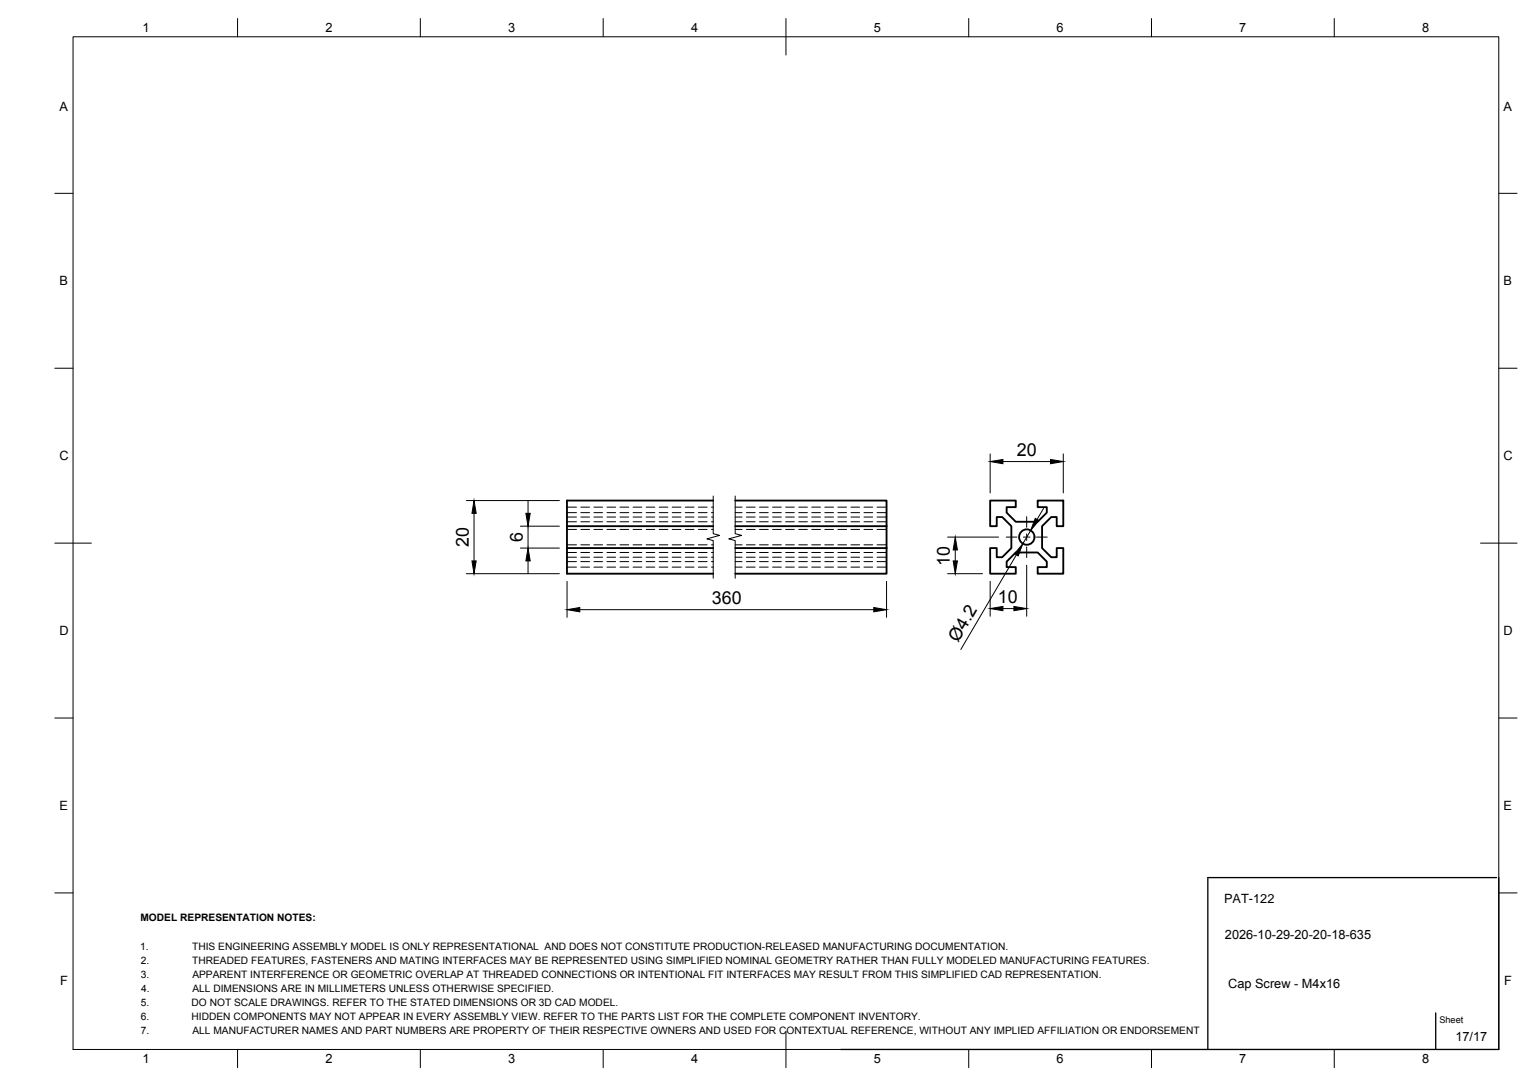
ISO-10303-21;
HEADER;
/* Generated by software containing ST-Developer
 * from STEP Tools, Inc. (www.steptools.com) 
 */

FILE_DESCRIPTION(
/* description */ ('PAT-122'),
/* implementation_level */ '2;1');

FILE_NAME(
/* name */ 'Cap Screw - M4x16.step',
/* time_stamp */ '2026-10-29T20:20:12-07:00',
/* author */ (''),
/* organization */ (''),
/* preprocessor_version */ 'ST-DEVELOPER v20.2',
/* originating_system */ 'Autodesk Translation Framework v15.17.0.0',
/* authorisation */ '');

FILE_SCHEMA (('AUTOMOTIVE_DESIGN { 1 0 10303 214 3 1 1 }'));
ENDSEC;

DATA;
#10=MECHANICAL_DESIGN_GEOMETRIC_PRESENTATION_REPRESENTATION('',(#512),#10019);
#413=CONICAL_SURFACE('',#6306,0.325,0.785398163397448);
#414=CONICAL_SURFACE('',#6310,0.335,0.785398163397448);
#415=CONICAL_SURFACE('',#6314,0.21,0.463647609000806);
#416=CONICAL_SURFACE('',#6318,0.18,0.785398163397448);
#420=ORIENTED_CLOSED_SHELL('',*,#5638,.F.);
#424=BREP_WITH_VOIDS('Body1',#5637,(#420));
#468=SHAPE_REPRESENTATION_RELATIONSHIP('SRR','None',#10189,#490);
#490=ADVANCED_BREP_SHAPE_REPRESENTATION('',(#424),#10018);
#512=STYLED_ITEM('',(#10355),#424);
#608=FACE_BOUND('',#1474,.T.);
#814=PLANE('',#6304);
#815=PLANE('',#6312);
#816=PLANE('',#6320);
#817=PLANE('',#6321);
#818=PLANE('',#6322);
#819=PLANE('',#6323);
#820=PLANE('',#6324);
#821=PLANE('',#6325);
#822=PLANE('',#6326);
#823=PLANE('',#6327);
#824=PLANE('',#6328);
#1100=FACE_OUTER_BOUND('',#1469,.T.);
#1101=FACE_OUTER_BOUND('',#1470,.T.);
#1102=FACE_OUTER_BOUND('',#1471,.T.);
#1103=FACE_OUTER_BOUND('',#1472,.T.);
#1104=FACE_OUTER_BOUND('',#1473,.T.);
#1105=FACE_OUTER_BOUND('',#1475,.T.);
#1106=FACE_OUTER_BOUND('',#1476,.T.);
#1107=FACE_OUTER_BOUND('',#1477,.T.);
#1108=FACE_OUTER_BOUND('',#1478,.T.);
#1109=FACE_OUTER_BOUND('',#1479,.T.);
#1110=FACE_OUTER_BOUND('',#1480,.T.);
#1111=FACE_OUTER_BOUND('',#1481,.T.);
#1112=FACE_OUTER_BOUND('',#1482,.T.);
#1113=FACE_OUTER_BOUND('',#1483,.T.);
#1114=FACE_OUTER_BOUND('',#1484,.T.);
#1115=FACE_OUTER_BOUND('',#1485,.T.);
#1116=FACE_OUTER_BOUND('',#1486,.T.);
#1469=EDGE_LOOP('',(#5197));
#1470=EDGE_LOOP('',(#5198,#5199,#5200,#5201));
#1471=EDGE_LOOP('',(#5202,#5203,#5204,#5205));
#1472=EDGE_LOOP('',(#5206,#5207,#5208,#5209));
#1473=EDGE_LOOP('',(#5210));
#1474=EDGE_LOOP('',(#5211));
#1475=EDGE_LOOP('',(#5212,#5213,#5214,#5215));
#1476=EDGE_LOOP('',(#5216,#5217,#5218,#5219));
#1477=EDGE_LOOP('',(#5220,#5221,#5222,#5223));
#1478=EDGE_LOOP('',(#5224));
#1479=EDGE_LOOP('',(#5225,#5226,#5227,#5228));
#1480=EDGE_LOOP('',(#5229,#5230,#5231,#5232));
#1481=EDGE_LOOP('',(#5233,#5234,#5235,#5236));
#1482=EDGE_LOOP('',(#5237,#5238,#5239,#5240));
#1483=EDGE_LOOP('',(#5241,#5242,#5243,#5244));
#1484=EDGE_LOOP('',(#5245,#5246,#5247,#5248));
#1485=EDGE_LOOP('',(#5249,#5250,#5251,#5252,#5253,#5254));
#1486=EDGE_LOOP('',(#5255,#5256,#5257,#5258,#5259,#5260));
#2007=LINE('',#9812,#2551);
#2008=LINE('',#9816,#2552);
#2009=LINE('',#9820,#2553);
#2010=LINE('',#9827,#2554);
#2011=LINE('',#9831,#2555);
#2012=LINE('',#9835,#2556);
#2013=LINE('',#9840,#2557);
#2014=LINE('',#9842,#2558);
#2015=LINE('',#9844,#2559);
#2016=LINE('',#9845,#2560);
#2017=LINE('',#9848,#2561);
#2018=LINE('',#9850,#2562);
#2019=LINE('',#9851,#2563);
#2020=LINE('',#9854,#2564);
#2021=LINE('',#9856,#2565);
#2022=LINE('',#9857,#2566);
#2023=LINE('',#9860,#2567);
#2024=LINE('',#9862,#2568);
#2025=LINE('',#9863,#2569);
#2026=LINE('',#9866,#2570);
#2027=LINE('',#9868,#2571);
#2028=LINE('',#9869,#2572);
#2029=LINE('',#9871,#2573);
#2030=LINE('',#9872,#2574);
#2551=VECTOR('',#7798,0.325);
#2552=VECTOR('',#7803,0.35);
#2553=VECTOR('',#7808,0.335);
#2554=VECTOR('',#7817,0.21);
#2555=VECTOR('',#7822,0.2);
#2556=VECTOR('',#7827,0.18);
#2557=VECTOR('',#7832,1.);
#2558=VECTOR('',#7833,1.);
#2559=VECTOR('',#7834,1.);
#2560=VECTOR('',#7835,1.);
#2561=VECTOR('',#7838,1.);
#2562=VECTOR('',#7839,1.);
#2563=VECTOR('',#7840,1.);
#2564=VECTOR('',#7843,1.);
#2565=VECTOR('',#7844,1.);
#2566=VECTOR('',#7845,1.);
#2567=VECTOR('',#7848,1.);
#2568=VECTOR('',#7849,1.);
#2569=VECTOR('',#7850,1.);
#2570=VECTOR('',#7853,1.);
#2571=VECTOR('',#7854,1.);
#2572=VECTOR('',#7855,1.);
#2573=VECTOR('',#7858,1.);
#2574=VECTOR('',#7859,1.);
#2697=CIRCLE('',#6305,0.3);
#2698=CIRCLE('',#6307,0.35);
#2699=CIRCLE('',#6309,0.35);
#2700=CIRCLE('',#6311,0.32);
#2701=CIRCLE('',#6313,0.22);
#2702=CIRCLE('',#6315,0.1954);
#2703=CIRCLE('',#6317,0.1954);
#2704=CIRCLE('',#6319,0.16);
#3147=VERTEX_POINT('',#9807);
#3148=VERTEX_POINT('',#9810);
#3149=VERTEX_POINT('',#9814);
#3150=VERTEX_POINT('',#9818);
#3151=VERTEX_POINT('',#9822);
#3152=VERTEX_POINT('',#9825);
#3153=VERTEX_POINT('',#9829);
#3154=VERTEX_POINT('',#9833);
#3155=VERTEX_POINT('',#9838);
#3156=VERTEX_POINT('',#9839);
#3157=VERTEX_POINT('',#9841);
#3158=VERTEX_POINT('',#9843);
#3159=VERTEX_POINT('',#9847);
#3160=VERTEX_POINT('',#9849);
#3161=VERTEX_POINT('',#9853);
#3162=VERTEX_POINT('',#9855);
#3163=VERTEX_POINT('',#9859);
#3164=VERTEX_POINT('',#9861);
#3165=VERTEX_POINT('',#9865);
#3166=VERTEX_POINT('',#9867);
#3833=EDGE_CURVE('',#3147,#3147,#2697,.T.);
#3834=EDGE_CURVE('',#3148,#3148,#2698,.T.);
#3835=EDGE_CURVE('',#3148,#3147,#2007,.T.);
#3836=EDGE_CURVE('',#3149,#3149,#2699,.T.);
#3837=EDGE_CURVE('',#3149,#3148,#2008,.T.);
#3838=EDGE_CURVE('',#3150,#3150,#2700,.T.);
#3839=EDGE_CURVE('',#3150,#3149,#2009,.T.);
#3840=EDGE_CURVE('',#3151,#3151,#2701,.T.);
#3841=EDGE_CURVE('',#3152,#3152,#2702,.F.);
#3842=EDGE_CURVE('',#3152,#3151,#2010,.T.);
#3843=EDGE_CURVE('',#3153,#3153,#2703,.F.);
#3844=EDGE_CURVE('',#3153,#3152,#2011,.T.);
#3845=EDGE_CURVE('',#3154,#3154,#2704,.T.);
#3846=EDGE_CURVE('',#3154,#3153,#2012,.T.);
#3847=EDGE_CURVE('',#3155,#3156,#2013,.T.);
#3848=EDGE_CURVE('',#3156,#3157,#2014,.T.);
#3849=EDGE_CURVE('',#3157,#3158,#2015,.T.);
#3850=EDGE_CURVE('',#3155,#3158,#2016,.T.);
#3851=EDGE_CURVE('',#3156,#3159,#2017,.T.);
#3852=EDGE_CURVE('',#3159,#3160,#2018,.T.);
#3853=EDGE_CURVE('',#3160,#3157,#2019,.T.);
#3854=EDGE_CURVE('',#3159,#3161,#2020,.T.);
#3855=EDGE_CURVE('',#3161,#3162,#2021,.T.);
#3856=EDGE_CURVE('',#3162,#3160,#2022,.T.);
#3857=EDGE_CURVE('',#3161,#3163,#2023,.T.);
#3858=EDGE_CURVE('',#3163,#3164,#2024,.T.);
#3859=EDGE_CURVE('',#3164,#3162,#2025,.T.);
#3860=EDGE_CURVE('',#3163,#3165,#2026,.T.);
#3861=EDGE_CURVE('',#3165,#3166,#2027,.T.);
#3862=EDGE_CURVE('',#3166,#3164,#2028,.T.);
#3863=EDGE_CURVE('',#3165,#3155,#2029,.T.);
#3864=EDGE_CURVE('',#3158,#3166,#2030,.T.);
#5197=ORIENTED_EDGE('',*,*,#3833,.F.);
#5198=ORIENTED_EDGE('',*,*,#3834,.F.);
#5199=ORIENTED_EDGE('',*,*,#3835,.T.);
#5200=ORIENTED_EDGE('',*,*,#3833,.T.);
#5201=ORIENTED_EDGE('',*,*,#3835,.F.);
#5202=ORIENTED_EDGE('',*,*,#3836,.F.);
#5203=ORIENTED_EDGE('',*,*,#3837,.T.);
#5204=ORIENTED_EDGE('',*,*,#3834,.T.);
#5205=ORIENTED_EDGE('',*,*,#3837,.F.);
#5206=ORIENTED_EDGE('',*,*,#3838,.F.);
#5207=ORIENTED_EDGE('',*,*,#3839,.T.);
#5208=ORIENTED_EDGE('',*,*,#3836,.T.);
#5209=ORIENTED_EDGE('',*,*,#3839,.F.);
#5210=ORIENTED_EDGE('',*,*,#3838,.T.);
#5211=ORIENTED_EDGE('',*,*,#3840,.F.);
#5212=ORIENTED_EDGE('',*,*,#3841,.F.);
#5213=ORIENTED_EDGE('',*,*,#3842,.T.);
#5214=ORIENTED_EDGE('',*,*,#3840,.T.);
#5215=ORIENTED_EDGE('',*,*,#3842,.F.);
#5216=ORIENTED_EDGE('',*,*,#3843,.F.);
#5217=ORIENTED_EDGE('',*,*,#3844,.T.);
#5218=ORIENTED_EDGE('',*,*,#3841,.T.);
#5219=ORIENTED_EDGE('',*,*,#3844,.F.);
#5220=ORIENTED_EDGE('',*,*,#3845,.F.);
#5221=ORIENTED_EDGE('',*,*,#3846,.T.);
#5222=ORIENTED_EDGE('',*,*,#3843,.T.);
#5223=ORIENTED_EDGE('',*,*,#3846,.F.);
#5224=ORIENTED_EDGE('',*,*,#3845,.T.);
#5225=ORIENTED_EDGE('',*,*,#3847,.T.);
#5226=ORIENTED_EDGE('',*,*,#3848,.T.);
#5227=ORIENTED_EDGE('',*,*,#3849,.T.);
#5228=ORIENTED_EDGE('',*,*,#3850,.F.);
#5229=ORIENTED_EDGE('',*,*,#3851,.T.);
#5230=ORIENTED_EDGE('',*,*,#3852,.T.);
#5231=ORIENTED_EDGE('',*,*,#3853,.T.);
#5232=ORIENTED_EDGE('',*,*,#3848,.F.);
#5233=ORIENTED_EDGE('',*,*,#3854,.T.);
#5234=ORIENTED_EDGE('',*,*,#3855,.T.);
#5235=ORIENTED_EDGE('',*,*,#3856,.T.);
#5236=ORIENTED_EDGE('',*,*,#3852,.F.);
#5237=ORIENTED_EDGE('',*,*,#3857,.T.);
#5238=ORIENTED_EDGE('',*,*,#3858,.T.);
#5239=ORIENTED_EDGE('',*,*,#3859,.T.);
#5240=ORIENTED_EDGE('',*,*,#3855,.F.);
#5241=ORIENTED_EDGE('',*,*,#3860,.T.);
#5242=ORIENTED_EDGE('',*,*,#3861,.T.);
#5243=ORIENTED_EDGE('',*,*,#3862,.T.);
#5244=ORIENTED_EDGE('',*,*,#3858,.F.);
#5245=ORIENTED_EDGE('',*,*,#3863,.T.);
#5246=ORIENTED_EDGE('',*,*,#3850,.T.);
#5247=ORIENTED_EDGE('',*,*,#3864,.T.);
#5248=ORIENTED_EDGE('',*,*,#3861,.F.);
#5249=ORIENTED_EDGE('',*,*,#3863,.F.);
#5250=ORIENTED_EDGE('',*,*,#3860,.F.);
#5251=ORIENTED_EDGE('',*,*,#3857,.F.);
#5252=ORIENTED_EDGE('',*,*,#3854,.F.);
#5253=ORIENTED_EDGE('',*,*,#3851,.F.);
#5254=ORIENTED_EDGE('',*,*,#3847,.F.);
#5255=ORIENTED_EDGE('',*,*,#3864,.F.);
#5256=ORIENTED_EDGE('',*,*,#3849,.F.);
#5257=ORIENTED_EDGE('',*,*,#3853,.F.);
#5258=ORIENTED_EDGE('',*,*,#3856,.F.);
#5259=ORIENTED_EDGE('',*,*,#3859,.F.);
#5260=ORIENTED_EDGE('',*,*,#3862,.F.);
#5319=CYLINDRICAL_SURFACE('',#6308,0.35);
#5320=CYLINDRICAL_SURFACE('',#6316,0.1954);
#5596=ADVANCED_FACE('',(#1100),#814,.T.);
#5597=ADVANCED_FACE('',(#1101),#413,.T.);
#5598=ADVANCED_FACE('',(#1102),#5319,.T.);
#5599=ADVANCED_FACE('',(#1103),#414,.T.);
#5600=ADVANCED_FACE('',(#1104,#608),#815,.T.);
#5601=ADVANCED_FACE('',(#1105),#415,.T.);
#5602=ADVANCED_FACE('',(#1106),#5320,.T.);
#5603=ADVANCED_FACE('',(#1107),#416,.T.);
#5604=ADVANCED_FACE('',(#1108),#816,.T.);
#5605=ADVANCED_FACE('',(#1109),#817,.F.);
#5606=ADVANCED_FACE('',(#1110),#818,.F.);
#5607=ADVANCED_FACE('',(#1111),#819,.F.);
#5608=ADVANCED_FACE('',(#1112),#820,.F.);
#5609=ADVANCED_FACE('',(#1113),#821,.F.);
#5610=ADVANCED_FACE('',(#1114),#822,.F.);
#5611=ADVANCED_FACE('',(#1115),#823,.F.);
#5612=ADVANCED_FACE('',(#1116),#824,.F.);
#5637=CLOSED_SHELL('',(#5596,#5597,#5598,#5599,#5600,#5601,#5602,#5603,
#5604));
#5638=CLOSED_SHELL('',(#5605,#5606,#5607,#5608,#5609,#5610,#5611,#5612));
#6303=AXIS2_PLACEMENT_3D('',#9805,#7788,#7789);
#6304=AXIS2_PLACEMENT_3D('',#9806,#7790,#7791);
#6305=AXIS2_PLACEMENT_3D('',#9808,#7792,#7793);
#6306=AXIS2_PLACEMENT_3D('',#9809,#7794,#7795);
#6307=AXIS2_PLACEMENT_3D('',#9811,#7796,#7797);
#6308=AXIS2_PLACEMENT_3D('',#9813,#7799,#7800);
#6309=AXIS2_PLACEMENT_3D('',#9815,#7801,#7802);
#6310=AXIS2_PLACEMENT_3D('',#9817,#7804,#7805);
#6311=AXIS2_PLACEMENT_3D('',#9819,#7806,#7807);
#6312=AXIS2_PLACEMENT_3D('',#9821,#7809,#7810);
#6313=AXIS2_PLACEMENT_3D('',#9823,#7811,#7812);
#6314=AXIS2_PLACEMENT_3D('',#9824,#7813,#7814);
#6315=AXIS2_PLACEMENT_3D('',#9826,#7815,#7816);
#6316=AXIS2_PLACEMENT_3D('',#9828,#7818,#7819);
#6317=AXIS2_PLACEMENT_3D('',#9830,#7820,#7821);
#6318=AXIS2_PLACEMENT_3D('',#9832,#7823,#7824);
#6319=AXIS2_PLACEMENT_3D('',#9834,#7825,#7826);
#6320=AXIS2_PLACEMENT_3D('',#9836,#7828,#7829);
#6321=AXIS2_PLACEMENT_3D('',#9837,#7830,#7831);
#6322=AXIS2_PLACEMENT_3D('',#9846,#7836,#7837);
#6323=AXIS2_PLACEMENT_3D('',#9852,#7841,#7842);
#6324=AXIS2_PLACEMENT_3D('',#9858,#7846,#7847);
#6325=AXIS2_PLACEMENT_3D('',#9864,#7851,#7852);
#6326=AXIS2_PLACEMENT_3D('',#9870,#7856,#7857);
#6327=AXIS2_PLACEMENT_3D('',#9873,#7860,#7861);
#6328=AXIS2_PLACEMENT_3D('',#9874,#7862,#7863);
#7788=DIRECTION('axis',(0.,0.,1.));
#7789=DIRECTION('refdir',(1.,0.,0.));
#7790=DIRECTION('center_axis',(0.,1.,0.));
#7791=DIRECTION('ref_axis',(0.,0.,1.));
#7792=DIRECTION('center_axis',(0.,-1.,0.));
#7793=DIRECTION('ref_axis',(1.,0.,0.));
#7794=DIRECTION('center_axis',(0.,-1.,0.));
#7795=DIRECTION('ref_axis',(1.,0.,0.));
#7796=DIRECTION('center_axis',(0.,-1.,0.));
#7797=DIRECTION('ref_axis',(1.,0.,0.));
#7798=DIRECTION('',(0.707106781186547,0.707106781186548,8.65956056235493E-17));
#7799=DIRECTION('center_axis',(0.,-1.,0.));
#7800=DIRECTION('ref_axis',(1.,0.,0.));
#7801=DIRECTION('center_axis',(0.,-1.,0.));
#7802=DIRECTION('ref_axis',(1.,0.,0.));
#7803=DIRECTION('',(0.,1.,0.));
#7804=DIRECTION('center_axis',(0.,1.,0.));
#7805=DIRECTION('ref_axis',(1.,0.,0.));
#7806=DIRECTION('center_axis',(0.,-1.,0.));
#7807=DIRECTION('ref_axis',(1.,0.,0.));
#7808=DIRECTION('',(-0.707106781186547,0.707106781186548,-8.65956056235493E-17));
#7809=DIRECTION('center_axis',(0.,-1.,0.));
#7810=DIRECTION('ref_axis',(0.,0.,-1.));
#7811=DIRECTION('center_axis',(0.,-1.,0.));
#7812=DIRECTION('ref_axis',(1.,0.,0.));
#7813=DIRECTION('center_axis',(0.,1.,0.));
#7814=DIRECTION('ref_axis',(1.,0.,0.));
#7815=DIRECTION('center_axis',(0.,1.,0.));
#7816=DIRECTION('ref_axis',(1.,0.,0.));
#7817=DIRECTION('',(-0.447213595499958,0.894427190999916,-5.47678698264203E-17));
#7818=DIRECTION('center_axis',(0.,-1.,0.));
#7819=DIRECTION('ref_axis',(1.,0.,0.));
#7820=DIRECTION('center_axis',(0.,1.,0.));
#7821=DIRECTION('ref_axis',(1.,0.,0.));
#7822=DIRECTION('',(0.,1.,0.));
#7823=DIRECTION('center_axis',(0.,1.,0.));
#7824=DIRECTION('ref_axis',(1.,0.,0.));
#7825=DIRECTION('center_axis',(0.,-1.,0.));
#7826=DIRECTION('ref_axis',(1.,0.,0.));
#7827=DIRECTION('',(-0.707106781186547,0.707106781186548,-8.65956056235493E-17));
#7828=DIRECTION('center_axis',(0.,-1.,0.));
#7829=DIRECTION('ref_axis',(0.,0.,-1.));
#7830=DIRECTION('center_axis',(0.866025403784439,0.,-0.5));
#7831=DIRECTION('ref_axis',(0.5,0.,0.866025403784439));
#7832=DIRECTION('',(-0.5,0.,-0.866025403784439));
#7833=DIRECTION('',(0.,-1.,0.));
#7834=DIRECTION('',(0.5,0.,0.866025403784439));
#7835=DIRECTION('',(0.,-1.,0.));
#7836=DIRECTION('center_axis',(1.60246890531964E-16,0.,-1.));
#7837=DIRECTION('ref_axis',(1.,0.,1.60246890531964E-16));
#7838=DIRECTION('',(-1.,0.,-1.60246890531964E-16));
#7839=DIRECTION('',(0.,-1.,0.));
#7840=DIRECTION('',(1.,0.,1.60246890531964E-16));
#7841=DIRECTION('center_axis',(-0.866025403784439,0.,-0.5));
#7842=DIRECTION('ref_axis',(0.5,0.,-0.866025403784439));
#7843=DIRECTION('',(-0.5,0.,0.866025403784439));
#7844=DIRECTION('',(0.,-1.,0.));
#7845=DIRECTION('',(0.5,0.,-0.866025403784439));
#7846=DIRECTION('center_axis',(-0.866025403784439,0.,0.5));
#7847=DIRECTION('ref_axis',(-0.5,0.,-0.866025403784439));
#7848=DIRECTION('',(0.5,0.,0.866025403784439));
#7849=DIRECTION('',(0.,-1.,0.));
#7850=DIRECTION('',(-0.5,0.,-0.866025403784439));
#7851=DIRECTION('center_axis',(-1.60246890531964E-16,0.,1.));
#7852=DIRECTION('ref_axis',(-1.,0.,-1.60246890531964E-16));
#7853=DIRECTION('',(1.,0.,1.60246890531964E-16));
#7854=DIRECTION('',(0.,-1.,0.));
#7855=DIRECTION('',(-1.,0.,-1.60246890531964E-16));
#7856=DIRECTION('center_axis',(0.866025403784439,0.,0.5));
#7857=DIRECTION('ref_axis',(-0.5,0.,0.866025403784439));
#7858=DIRECTION('',(0.5,0.,-0.866025403784439));
#7859=DIRECTION('',(-0.5,0.,0.866025403784439));
#7860=DIRECTION('center_axis',(0.,1.,0.));
#7861=DIRECTION('ref_axis',(1.,0.,0.));
#7862=DIRECTION('center_axis',(0.,-1.,0.));
#7863=DIRECTION('ref_axis',(0.,0.,-1.));
#9805=CARTESIAN_POINT('',(0.,0.,0.));
#9806=CARTESIAN_POINT('Origin',(0.3,0.4,0.));
#9807=CARTESIAN_POINT('',(-0.3,0.4,-3.67394039744206E-17));
#9808=CARTESIAN_POINT('Origin',(0.,0.4,0.));
#9809=CARTESIAN_POINT('Origin',(0.,0.375,0.));
#9810=CARTESIAN_POINT('',(-0.35,0.35,-4.28626379701573E-17));
#9811=CARTESIAN_POINT('Origin',(0.,0.35,0.));
#9812=CARTESIAN_POINT('',(-0.325,0.375,-3.9801020972289E-17));
#9813=CARTESIAN_POINT('Origin',(0.,0.19,0.));
#9814=CARTESIAN_POINT('',(-0.35,0.03,-4.28626379701574E-17));
#9815=CARTESIAN_POINT('Origin',(0.,0.03,0.));
#9816=CARTESIAN_POINT('',(-0.35,0.19,-4.28626379701574E-17));
#9817=CARTESIAN_POINT('Origin',(0.,0.0149999999999999,0.));
#9818=CARTESIAN_POINT('',(-0.32,-3.29597460435593E-17,-3.91886975727153E-17));
#9819=CARTESIAN_POINT('Origin',(0.,0.,0.));
#9820=CARTESIAN_POINT('',(-0.335,0.0149999999999999,-4.10256677714363E-17));
#9821=CARTESIAN_POINT('Origin',(0.22,0.,0.));
#9822=CARTESIAN_POINT('',(-0.22,-6.93889390390723E-18,-2.69422295812418E-17));
#9823=CARTESIAN_POINT('Origin',(0.,0.,0.));
#9824=CARTESIAN_POINT('Origin',(0.,-0.02,0.));
#9825=CARTESIAN_POINT('',(-0.1954,-0.0492,2.39295984553393E-17));
#9826=CARTESIAN_POINT('Origin',(0.,-0.0492,0.));
#9827=CARTESIAN_POINT('',(-0.21,-0.02,-2.57175827820944E-17));
#9828=CARTESIAN_POINT('Origin',(0.,-0.8,0.));
#9829=CARTESIAN_POINT('',(-0.1954,-1.5646,2.39295984553393E-17));
#9830=CARTESIAN_POINT('Origin',(0.,-1.5646,0.));
#9831=CARTESIAN_POINT('',(-0.1954,-0.8,-2.39295984553393E-17));
#9832=CARTESIAN_POINT('Origin',(0.,-1.58,0.));
#9833=CARTESIAN_POINT('',(-0.16,-1.6,-1.95943487863577E-17));
#9834=CARTESIAN_POINT('Origin',(0.,-1.6,0.));
#9835=CARTESIAN_POINT('',(-0.18,-1.58,-2.20436423846524E-17));
#9836=CARTESIAN_POINT('Origin',(0.,-1.6,0.));
#9837=CARTESIAN_POINT('Origin',(0.0866025403784439,-0.4,-0.15));
#9838=CARTESIAN_POINT('',(0.173205080756888,-0.4,0.));
#9839=CARTESIAN_POINT('',(0.0866025403784439,-0.4,-0.15));
#9840=CARTESIAN_POINT('',(0.173205080756888,-0.4,0.));
#9841=CARTESIAN_POINT('',(0.0866025403784439,-0.64,-0.15));
#9842=CARTESIAN_POINT('',(0.0866025403784439,-0.4,-0.15));
#9843=CARTESIAN_POINT('',(0.173205080756888,-0.64,0.));
#9844=CARTESIAN_POINT('',(0.173205080756888,-0.64,0.));
#9845=CARTESIAN_POINT('',(0.173205080756888,-0.4,0.));
#9846=CARTESIAN_POINT('Origin',(-0.0866025403784438,-0.4,-0.15));
#9847=CARTESIAN_POINT('',(-0.0866025403784438,-0.4,-0.15));
#9848=CARTESIAN_POINT('',(0.0866025403784439,-0.4,-0.15));
#9849=CARTESIAN_POINT('',(-0.0866025403784438,-0.64,-0.15));
#9850=CARTESIAN_POINT('',(-0.0866025403784438,-0.4,-0.15));
#9851=CARTESIAN_POINT('',(0.0866025403784439,-0.64,-0.15));
#9852=CARTESIAN_POINT('Origin',(-0.173205080756888,-0.4,-2.77555756156289E-17));
#9853=CARTESIAN_POINT('',(-0.173205080756888,-0.4,-2.12115047744981E-17));
#9854=CARTESIAN_POINT('',(-0.0866025403784438,-0.4,-0.15));
#9855=CARTESIAN_POINT('',(-0.173205080756888,-0.64,-2.77555756156289E-17));
#9856=CARTESIAN_POINT('',(-0.173205080756888,-0.4,-2.12115047744981E-17));
#9857=CARTESIAN_POINT('',(-0.0866025403784438,-0.64,-0.15));
#9858=CARTESIAN_POINT('Origin',(-0.0866025403784439,-0.4,0.15));
#9859=CARTESIAN_POINT('',(-0.0866025403784439,-0.4,0.15));
#9860=CARTESIAN_POINT('',(-0.173205080756888,-0.4,-2.12115047744981E-17));
#9861=CARTESIAN_POINT('',(-0.0866025403784439,-0.64,0.15));
#9862=CARTESIAN_POINT('',(-0.0866025403784439,-0.4,0.15));
#9863=CARTESIAN_POINT('',(-0.173205080756888,-0.64,-2.12115047744981E-17));
#9864=CARTESIAN_POINT('Origin',(0.0866025403784439,-0.4,0.15));
#9865=CARTESIAN_POINT('',(0.0866025403784439,-0.4,0.15));
#9866=CARTESIAN_POINT('',(-0.0866025403784439,-0.4,0.15));
#9867=CARTESIAN_POINT('',(0.0866025403784439,-0.64,0.15));
#9868=CARTESIAN_POINT('',(0.0866025403784439,-0.4,0.15));
#9869=CARTESIAN_POINT('',(-0.0866025403784439,-0.64,0.15));
#9870=CARTESIAN_POINT('Origin',(0.173205080756888,-0.4,0.));
#9871=CARTESIAN_POINT('',(0.0866025403784439,-0.4,0.15));
#9872=CARTESIAN_POINT('',(0.0866025403784439,-0.64,0.15));
#9873=CARTESIAN_POINT('Origin',(0.,-0.4,-2.77555756156289E-17));
#9874=CARTESIAN_POINT('Origin',(0.,-0.64,-2.77555756156289E-17));
#9994=UNCERTAINTY_MEASURE_WITH_UNIT(LENGTH_MEASURE(0.001),#10020,
'DISTANCE_ACCURACY_VALUE',
'Maximum model space distance between geometric entities at asserted c
onnectivities');
#9995=UNCERTAINTY_MEASURE_WITH_UNIT(LENGTH_MEASURE(0.001),#10020,
'DISTANCE_ACCURACY_VALUE',
'Maximum model space distance between geometric entities at asserted c
onnectivities');
#10018=(
GEOMETRIC_REPRESENTATION_CONTEXT(3)
GLOBAL_UNCERTAINTY_ASSIGNED_CONTEXT((#9994))
GLOBAL_UNIT_ASSIGNED_CONTEXT((#10020,#10022,#10023))
REPRESENTATION_CONTEXT('','3D')
);
#10019=(
GEOMETRIC_REPRESENTATION_CONTEXT(3)
GLOBAL_UNCERTAINTY_ASSIGNED_CONTEXT((#9995))
GLOBAL_UNIT_ASSIGNED_CONTEXT((#10020,#10022,#10023))
REPRESENTATION_CONTEXT('','3D')
);
#10020=(
LENGTH_UNIT()
NAMED_UNIT(*)
SI_UNIT(.CENTI.,.METRE.)
);
#10022=(
NAMED_UNIT(*)
PLANE_ANGLE_UNIT()
SI_UNIT($,.RADIAN.)
);
#10023=(
NAMED_UNIT(*)
SI_UNIT($,.STERADIAN.)
SOLID_ANGLE_UNIT()
);
#10046=SHAPE_DEFINITION_REPRESENTATION(#10069,#10189);
#10069=PRODUCT_DEFINITION_SHAPE('',$,#10213);
#10189=SHAPE_REPRESENTATION('',(#6303),#10018);
#10190=PRODUCT_DEFINITION_CONTEXT('part definition',#10261,'design');
#10213=PRODUCT_DEFINITION('Cap Screw - M4x16',
'Cap Screw - M4x16',#10236,#10190);
#10236=PRODUCT_DEFINITION_FORMATION('',$,#10285);
#10261=APPLICATION_CONTEXT(
'Core Data for Automotive Mechanical Design Process');
#10262=PRODUCT_CONTEXT('part definition',#10261,'mechanical');
#10285=PRODUCT('Cap Screw - M4x16','Cap Screw - M4x16',
'Cap Screw - M4x16',(#10262));
#10349=COLOUR_RGB('Black',0.12,0.14,0.17);
#10350=FILL_AREA_STYLE_COLOUR('',#10349);
#10351=FILL_AREA_STYLE('',(#10350));
#10352=SURFACE_STYLE_FILL_AREA(#10351);
#10353=SURFACE_SIDE_STYLE('',(#10352));
#10354=SURFACE_STYLE_USAGE(.BOTH.,#10353);
#10355=PRESENTATION_STYLE_ASSIGNMENT((#10354));
ENDSEC;
END-ISO-10303-21;
